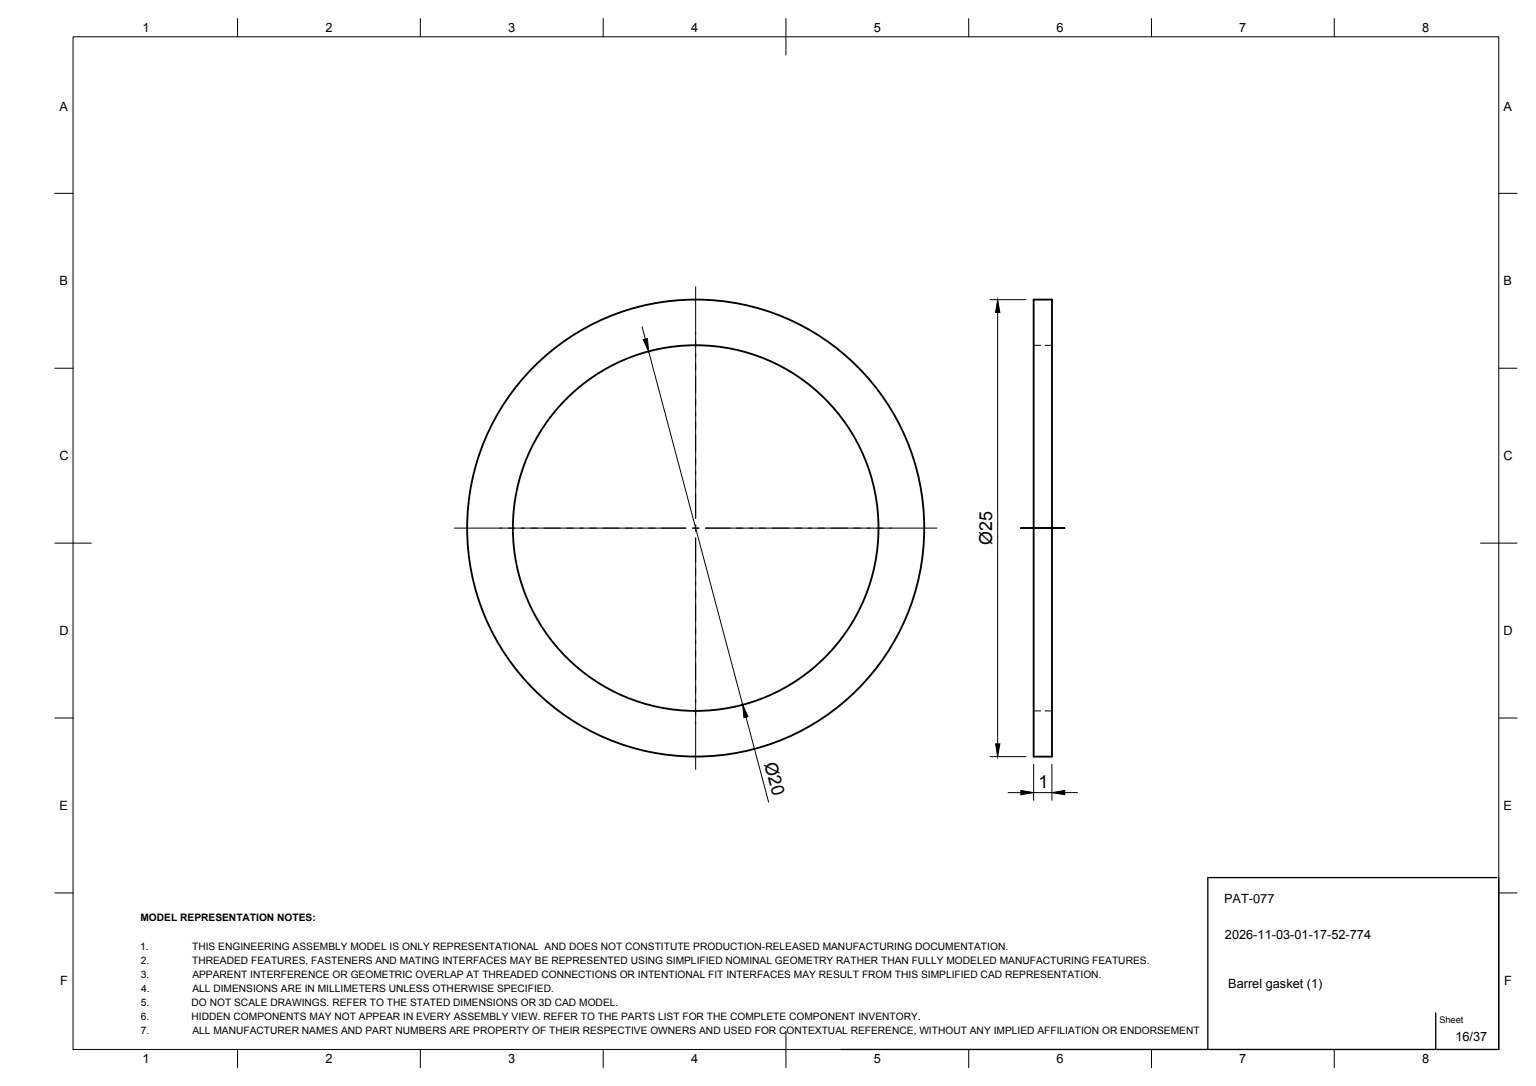
ISO-10303-21;
HEADER;
/* Generated by software containing ST-Developer
 * from STEP Tools, Inc. (www.steptools.com) 
 */

FILE_DESCRIPTION(
/* description */ ('Pallet stop with pneumatic fitting'),
/* implementation_level */ '2;1');

FILE_NAME(
/* name */ 'Barrel gasket (1).step',
/* time_stamp */ '2026-10-27T10:51:41-07:00',
/* author */ (''),
/* organization */ (''),
/* preprocessor_version */ 'ST-DEVELOPER v20.2',
/* originating_system */ 'Autodesk Translation Framework v15.17.0.0',
/* authorisation */ '');

FILE_SCHEMA (('AUTOMOTIVE_DESIGN { 1 0 10303 214 3 1 1 }'));
ENDSEC;

DATA;
#10=MECHANICAL_DESIGN_GEOMETRIC_PRESENTATION_REPRESENTATION('',(#368),#10265);
#304=SHAPE_REPRESENTATION_RELATIONSHIP('SRR','None',#10417,#336);
#336=ADVANCED_BREP_SHAPE_REPRESENTATION('',(#400),#10241);
#368=STYLED_ITEM('',(#10641),#400);
#400=MANIFOLD_SOLID_BREP('Body1',#5056);
#498=FACE_BOUND('',#1266,.T.);
#499=FACE_BOUND('',#1268,.T.);
#618=PLANE('',#5707);
#619=PLANE('',#5708);
#870=FACE_OUTER_BOUND('',#1263,.T.);
#871=FACE_OUTER_BOUND('',#1264,.T.);
#872=FACE_OUTER_BOUND('',#1265,.T.);
#873=FACE_OUTER_BOUND('',#1267,.T.);
#1263=EDGE_LOOP('',(#3940,#3941,#3942,#3943));
#1264=EDGE_LOOP('',(#3944,#3945,#3946,#3947));
#1265=EDGE_LOOP('',(#3948));
#1266=EDGE_LOOP('',(#3949));
#1267=EDGE_LOOP('',(#3950));
#1268=EDGE_LOOP('',(#3951));
#1626=LINE('',#9283,#1961);
#1627=LINE('',#9289,#1962);
#1961=VECTOR('',#6767,1.);
#1962=VECTOR('',#6774,1.25);
#2282=CIRCLE('',#5702,1.);
#2283=CIRCLE('',#5703,1.);
#2284=CIRCLE('',#5705,1.25);
#2285=CIRCLE('',#5706,1.25);
#2582=VERTEX_POINT('',#9280);
#2583=VERTEX_POINT('',#9282);
#2584=VERTEX_POINT('',#9286);
#2585=VERTEX_POINT('',#9288);
#3069=EDGE_CURVE('',#2582,#2582,#2282,.T.);
#3070=EDGE_CURVE('',#2582,#2583,#1626,.T.);
#3071=EDGE_CURVE('',#2583,#2583,#2283,.T.);
#3072=EDGE_CURVE('',#2584,#2584,#2284,.T.);
#3073=EDGE_CURVE('',#2584,#2585,#1627,.T.);
#3074=EDGE_CURVE('',#2585,#2585,#2285,.T.);
#3940=ORIENTED_EDGE('',*,*,#3069,.F.);
#3941=ORIENTED_EDGE('',*,*,#3070,.T.);
#3942=ORIENTED_EDGE('',*,*,#3071,.T.);
#3943=ORIENTED_EDGE('',*,*,#3070,.F.);
#3944=ORIENTED_EDGE('',*,*,#3072,.F.);
#3945=ORIENTED_EDGE('',*,*,#3073,.T.);
#3946=ORIENTED_EDGE('',*,*,#3074,.T.);
#3947=ORIENTED_EDGE('',*,*,#3073,.F.);
#3948=ORIENTED_EDGE('',*,*,#3072,.T.);
#3949=ORIENTED_EDGE('',*,*,#3069,.T.);
#3950=ORIENTED_EDGE('',*,*,#3074,.F.);
#3951=ORIENTED_EDGE('',*,*,#3071,.F.);
#4682=CYLINDRICAL_SURFACE('',#5701,1.);
#4683=CYLINDRICAL_SURFACE('',#5704,1.25);
#4865=ADVANCED_FACE('',(#870),#4682,.F.);
#4866=ADVANCED_FACE('',(#871),#4683,.T.);
#4867=ADVANCED_FACE('',(#872,#498),#618,.T.);
#4868=ADVANCED_FACE('',(#873,#499),#619,.F.);
#5056=CLOSED_SHELL('',(#4865,#4866,#4867,#4868));
#5700=AXIS2_PLACEMENT_3D('',#9278,#6761,#6762);
#5701=AXIS2_PLACEMENT_3D('',#9279,#6763,#6764);
#5702=AXIS2_PLACEMENT_3D('',#9281,#6765,#6766);
#5703=AXIS2_PLACEMENT_3D('',#9284,#6768,#6769);
#5704=AXIS2_PLACEMENT_3D('',#9285,#6770,#6771);
#5705=AXIS2_PLACEMENT_3D('',#9287,#6772,#6773);
#5706=AXIS2_PLACEMENT_3D('',#9290,#6775,#6776);
#5707=AXIS2_PLACEMENT_3D('',#9291,#6777,#6778);
#5708=AXIS2_PLACEMENT_3D('',#9292,#6779,#6780);
#6761=DIRECTION('axis',(0.,0.,1.));
#6762=DIRECTION('refdir',(1.,0.,0.));
#6763=DIRECTION('center_axis',(0.,0.,1.));
#6764=DIRECTION('ref_axis',(1.,0.,0.));
#6765=DIRECTION('center_axis',(0.,0.,-1.));
#6766=DIRECTION('ref_axis',(1.,0.,0.));
#6767=DIRECTION('',(0.,0.,-1.));
#6768=DIRECTION('center_axis',(0.,0.,-1.));
#6769=DIRECTION('ref_axis',(1.,0.,0.));
#6770=DIRECTION('center_axis',(0.,0.,1.));
#6771=DIRECTION('ref_axis',(1.,0.,0.));
#6772=DIRECTION('center_axis',(0.,0.,1.));
#6773=DIRECTION('ref_axis',(1.,0.,0.));
#6774=DIRECTION('',(0.,0.,-1.));
#6775=DIRECTION('center_axis',(0.,0.,1.));
#6776=DIRECTION('ref_axis',(1.,0.,0.));
#6777=DIRECTION('center_axis',(0.,0.,1.));
#6778=DIRECTION('ref_axis',(1.,0.,0.));
#6779=DIRECTION('center_axis',(0.,0.,1.));
#6780=DIRECTION('ref_axis',(1.,0.,0.));
#9278=CARTESIAN_POINT('',(0.,0.,0.));
#9279=CARTESIAN_POINT('Origin',(4.,4.,8.));
#9280=CARTESIAN_POINT('',(3.,4.,8.1));
#9281=CARTESIAN_POINT('Origin',(4.,4.,8.1));
#9282=CARTESIAN_POINT('',(3.,4.,8.));
#9283=CARTESIAN_POINT('',(3.,4.,8.));
#9284=CARTESIAN_POINT('Origin',(4.,4.,8.));
#9285=CARTESIAN_POINT('Origin',(4.,4.,8.));
#9286=CARTESIAN_POINT('',(2.75,4.,8.1));
#9287=CARTESIAN_POINT('Origin',(4.,4.,8.1));
#9288=CARTESIAN_POINT('',(2.75,4.,8.));
#9289=CARTESIAN_POINT('',(2.75,4.,8.));
#9290=CARTESIAN_POINT('Origin',(4.,4.,8.));
#9291=CARTESIAN_POINT('Origin',(4.,4.,8.1));
#9292=CARTESIAN_POINT('Origin',(4.,4.,8.));
#10203=UNCERTAINTY_MEASURE_WITH_UNIT(LENGTH_MEASURE(0.001),#10266,
'DISTANCE_ACCURACY_VALUE',
'Maximum model space distance between geometric entities at asserted c
onnectivities');
#10227=UNCERTAINTY_MEASURE_WITH_UNIT(LENGTH_MEASURE(0.001),#10266,
'DISTANCE_ACCURACY_VALUE',
'Maximum model space distance between geometric entities at asserted c
onnectivities');
#10241=(
GEOMETRIC_REPRESENTATION_CONTEXT(3)
GLOBAL_UNCERTAINTY_ASSIGNED_CONTEXT((#10203))
GLOBAL_UNIT_ASSIGNED_CONTEXT((#10266,#10268,#10269))
REPRESENTATION_CONTEXT('','3D')
);
#10265=(
GEOMETRIC_REPRESENTATION_CONTEXT(3)
GLOBAL_UNCERTAINTY_ASSIGNED_CONTEXT((#10227))
GLOBAL_UNIT_ASSIGNED_CONTEXT((#10266,#10268,#10269))
REPRESENTATION_CONTEXT('','3D')
);
#10266=(
LENGTH_UNIT()
NAMED_UNIT(*)
SI_UNIT(.CENTI.,.METRE.)
);
#10268=(
NAMED_UNIT(*)
PLANE_ANGLE_UNIT()
SI_UNIT($,.RADIAN.)
);
#10269=(
NAMED_UNIT(*)
SI_UNIT($,.STERADIAN.)
SOLID_ANGLE_UNIT()
);
#10283=SHAPE_DEFINITION_REPRESENTATION(#10320,#10417);
#10320=PRODUCT_DEFINITION_SHAPE('',$,#10455);
#10417=SHAPE_REPRESENTATION('',(#5700),#10241);
#10441=PRODUCT_DEFINITION_CONTEXT('part definition',#10554,'design');
#10455=PRODUCT_DEFINITION('Barrel gasket (1)','Barrel gasket (1)',#10492,
#10441);
#10492=PRODUCT_DEFINITION_FORMATION('',$,#10569);
#10554=APPLICATION_CONTEXT(
'Core Data for Automotive Mechanical Design Process');
#10555=PRODUCT_CONTEXT('part definition',#10554,'mechanical');
#10569=PRODUCT('Barrel gasket (1)','Barrel gasket (1)','Barrel gasket (1)',(#10555));
#10635=COLOUR_RGB('Light Blue',0.38,0.62,0.78);
#10636=FILL_AREA_STYLE_COLOUR('',#10635);
#10637=FILL_AREA_STYLE('',(#10636));
#10638=SURFACE_STYLE_FILL_AREA(#10637);
#10639=SURFACE_SIDE_STYLE('',(#10638));
#10640=SURFACE_STYLE_USAGE(.BOTH.,#10639);
#10641=PRESENTATION_STYLE_ASSIGNMENT((#10640));
ENDSEC;
END-ISO-10303-21;
